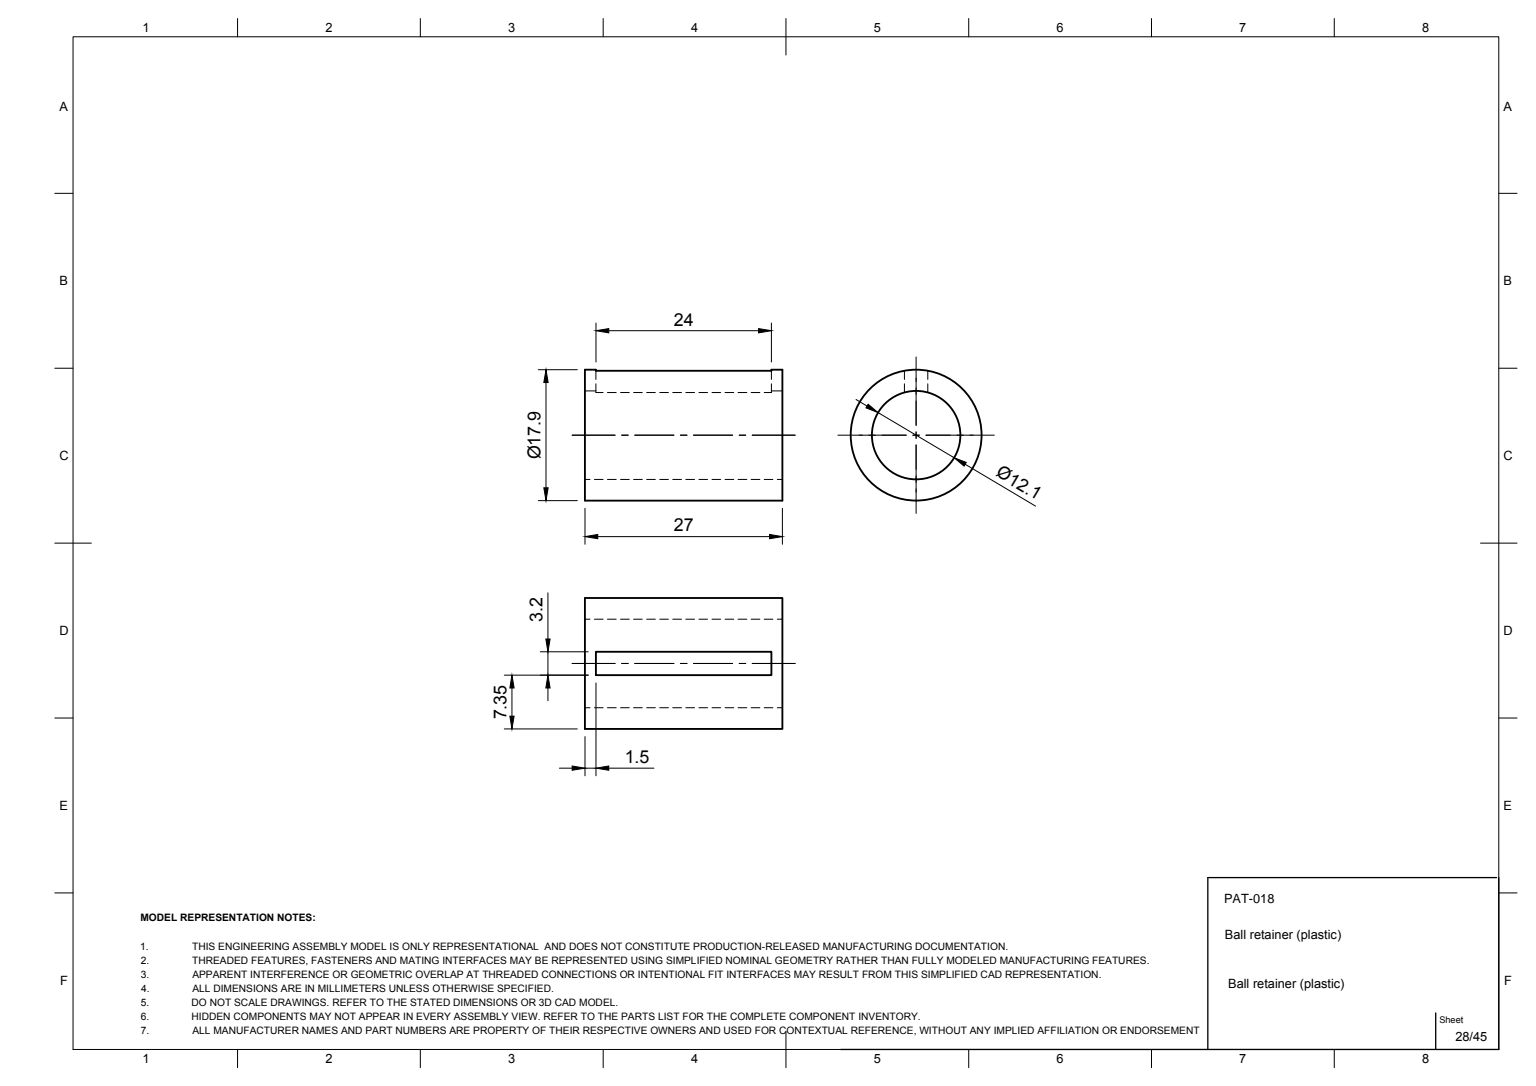
ISO-10303-21;
HEADER;
/* Generated by software containing ST-Developer
 * from STEP Tools, Inc. (www.steptools.com) 
 */

FILE_DESCRIPTION(
/* description */ ('Cam-driven reciprocating slide'),
/* implementation_level */ '2;1');

FILE_NAME(
/* name */ 'Ball retainer (plastic).step',
/* time_stamp */ '2026-10-28T03:25:20-07:00',
/* author */ (''),
/* organization */ (''),
/* preprocessor_version */ 'ST-DEVELOPER v20.2',
/* originating_system */ 'Autodesk Translation Framework v15.17.0.0',
/* authorisation */ '');

FILE_SCHEMA (('AUTOMOTIVE_DESIGN { 1 0 10303 214 3 1 1 }'));
ENDSEC;

DATA;
#10=MECHANICAL_DESIGN_GEOMETRIC_PRESENTATION_REPRESENTATION('',(#449),#13277);
#368=SHAPE_REPRESENTATION_RELATIONSHIP('SRR','None',#13463,#405);
#405=ADVANCED_BREP_SHAPE_REPRESENTATION('',(#492),#13258);
#449=STYLED_ITEM('',(#13713),#492);
#492=MANIFOLD_SOLID_BREP('Body1',#6426);
#635=FACE_BOUND('',#1646,.T.);
#636=FACE_BOUND('',#1648,.T.);
#637=FACE_BOUND('',#1650,.T.);
#638=FACE_BOUND('',#1652,.T.);
#802=PLANE('',#7342);
#803=PLANE('',#7345);
#804=PLANE('',#7346);
#805=PLANE('',#7349);
#806=PLANE('',#7350);
#807=PLANE('',#7355);
#1134=FACE_OUTER_BOUND('',#1641,.T.);
#1135=FACE_OUTER_BOUND('',#1642,.T.);
#1136=FACE_OUTER_BOUND('',#1643,.T.);
#1137=FACE_OUTER_BOUND('',#1644,.T.);
#1138=FACE_OUTER_BOUND('',#1645,.T.);
#1139=FACE_OUTER_BOUND('',#1647,.T.);
#1140=FACE_OUTER_BOUND('',#1649,.T.);
#1141=FACE_OUTER_BOUND('',#1651,.T.);
#1641=EDGE_LOOP('',(#5330,#5331,#5332,#5333));
#1642=EDGE_LOOP('',(#5334,#5335,#5336,#5337));
#1643=EDGE_LOOP('',(#5338,#5339,#5340,#5341));
#1644=EDGE_LOOP('',(#5342,#5343,#5344,#5345));
#1645=EDGE_LOOP('',(#5346));
#1646=EDGE_LOOP('',(#5347));
#1647=EDGE_LOOP('',(#5348,#5349,#5350,#5351));
#1648=EDGE_LOOP('',(#5352,#5353,#5354,#5355));
#1649=EDGE_LOOP('',(#5356));
#1650=EDGE_LOOP('',(#5357));
#1651=EDGE_LOOP('',(#5358,#5359,#5360,#5361));
#1652=EDGE_LOOP('',(#5362,#5363,#5364,#5365));
#2088=LINE('',#12499,#2527);
#2089=LINE('',#12502,#2528);
#2090=LINE('',#12505,#2529);
#2091=LINE('',#12507,#2530);
#2092=LINE('',#12508,#2531);
#2093=LINE('',#12514,#2532);
#2094=LINE('',#12516,#2533);
#2095=LINE('',#12517,#2534);
#2096=LINE('',#12526,#2535);
#2097=LINE('',#12531,#2536);
#2527=VECTOR('',#8906,1.);
#2528=VECTOR('',#8909,1.);
#2529=VECTOR('',#8912,1.);
#2530=VECTOR('',#8913,1.);
#2531=VECTOR('',#8914,1.);
#2532=VECTOR('',#8921,1.);
#2533=VECTOR('',#8924,1.);
#2534=VECTOR('',#8925,1.);
#2535=VECTOR('',#8936,0.895);
#2536=VECTOR('',#8943,0.605);
#2938=CIRCLE('',#7343,0.895);
#2939=CIRCLE('',#7344,0.605);
#2940=CIRCLE('',#7347,0.895);
#2941=CIRCLE('',#7348,0.605);
#2942=CIRCLE('',#7351,0.895);
#2943=CIRCLE('',#7352,0.605);
#2944=CIRCLE('',#7354,0.895);
#2945=CIRCLE('',#7356,0.605);
#3373=VERTEX_POINT('',#12495);
#3374=VERTEX_POINT('',#12496);
#3375=VERTEX_POINT('',#12498);
#3376=VERTEX_POINT('',#12500);
#3377=VERTEX_POINT('',#12504);
#3378=VERTEX_POINT('',#12506);
#3379=VERTEX_POINT('',#12510);
#3380=VERTEX_POINT('',#12512);
#3381=VERTEX_POINT('',#12519);
#3382=VERTEX_POINT('',#12521);
#3383=VERTEX_POINT('',#12524);
#3384=VERTEX_POINT('',#12528);
#4055=EDGE_CURVE('',#3373,#3374,#2938,.T.);
#4056=EDGE_CURVE('',#3375,#3373,#2088,.T.);
#4057=EDGE_CURVE('',#3376,#3375,#2939,.T.);
#4058=EDGE_CURVE('',#3374,#3376,#2089,.T.);
#4059=EDGE_CURVE('',#3374,#3377,#2090,.T.);
#4060=EDGE_CURVE('',#3378,#3376,#2091,.T.);
#4061=EDGE_CURVE('',#3378,#3377,#2092,.T.);
#4062=EDGE_CURVE('',#3377,#3379,#2940,.T.);
#4063=EDGE_CURVE('',#3380,#3378,#2941,.T.);
#4064=EDGE_CURVE('',#3379,#3380,#2093,.T.);
#4065=EDGE_CURVE('',#3379,#3373,#2094,.T.);
#4066=EDGE_CURVE('',#3375,#3380,#2095,.T.);
#4067=EDGE_CURVE('',#3381,#3381,#2942,.T.);
#4068=EDGE_CURVE('',#3382,#3382,#2943,.T.);
#4069=EDGE_CURVE('',#3383,#3383,#2944,.T.);
#4070=EDGE_CURVE('',#3383,#3381,#2096,.T.);
#4071=EDGE_CURVE('',#3384,#3384,#2945,.T.);
#4072=EDGE_CURVE('',#3384,#3382,#2097,.T.);
#5330=ORIENTED_EDGE('',*,*,#4055,.F.);
#5331=ORIENTED_EDGE('',*,*,#4056,.F.);
#5332=ORIENTED_EDGE('',*,*,#4057,.F.);
#5333=ORIENTED_EDGE('',*,*,#4058,.F.);
#5334=ORIENTED_EDGE('',*,*,#4059,.F.);
#5335=ORIENTED_EDGE('',*,*,#4058,.T.);
#5336=ORIENTED_EDGE('',*,*,#4060,.F.);
#5337=ORIENTED_EDGE('',*,*,#4061,.T.);
#5338=ORIENTED_EDGE('',*,*,#4062,.F.);
#5339=ORIENTED_EDGE('',*,*,#4061,.F.);
#5340=ORIENTED_EDGE('',*,*,#4063,.F.);
#5341=ORIENTED_EDGE('',*,*,#4064,.F.);
#5342=ORIENTED_EDGE('',*,*,#4065,.F.);
#5343=ORIENTED_EDGE('',*,*,#4064,.T.);
#5344=ORIENTED_EDGE('',*,*,#4066,.F.);
#5345=ORIENTED_EDGE('',*,*,#4056,.T.);
#5346=ORIENTED_EDGE('',*,*,#4067,.F.);
#5347=ORIENTED_EDGE('',*,*,#4068,.T.);
#5348=ORIENTED_EDGE('',*,*,#4069,.F.);
#5349=ORIENTED_EDGE('',*,*,#4070,.T.);
#5350=ORIENTED_EDGE('',*,*,#4067,.T.);
#5351=ORIENTED_EDGE('',*,*,#4070,.F.);
#5352=ORIENTED_EDGE('',*,*,#4062,.T.);
#5353=ORIENTED_EDGE('',*,*,#4065,.T.);
#5354=ORIENTED_EDGE('',*,*,#4055,.T.);
#5355=ORIENTED_EDGE('',*,*,#4059,.T.);
#5356=ORIENTED_EDGE('',*,*,#4069,.T.);
#5357=ORIENTED_EDGE('',*,*,#4071,.F.);
#5358=ORIENTED_EDGE('',*,*,#4071,.T.);
#5359=ORIENTED_EDGE('',*,*,#4072,.T.);
#5360=ORIENTED_EDGE('',*,*,#4068,.F.);
#5361=ORIENTED_EDGE('',*,*,#4072,.F.);
#5362=ORIENTED_EDGE('',*,*,#4063,.T.);
#5363=ORIENTED_EDGE('',*,*,#4060,.T.);
#5364=ORIENTED_EDGE('',*,*,#4057,.T.);
#5365=ORIENTED_EDGE('',*,*,#4066,.T.);
#5979=CYLINDRICAL_SURFACE('',#7353,0.895);
#5980=CYLINDRICAL_SURFACE('',#7357,0.605);
#6252=ADVANCED_FACE('',(#1134),#802,.F.);
#6253=ADVANCED_FACE('',(#1135),#803,.F.);
#6254=ADVANCED_FACE('',(#1136),#804,.F.);
#6255=ADVANCED_FACE('',(#1137),#805,.F.);
#6256=ADVANCED_FACE('',(#1138,#635),#806,.T.);
#6257=ADVANCED_FACE('',(#1139,#636),#5979,.T.);
#6258=ADVANCED_FACE('',(#1140,#637),#807,.T.);
#6259=ADVANCED_FACE('',(#1141,#638),#5980,.F.);
#6426=CLOSED_SHELL('',(#6252,#6253,#6254,#6255,#6256,#6257,#6258,#6259));
#7341=AXIS2_PLACEMENT_3D('',#12493,#8900,#8901);
#7342=AXIS2_PLACEMENT_3D('',#12494,#8902,#8903);
#7343=AXIS2_PLACEMENT_3D('',#12497,#8904,#8905);
#7344=AXIS2_PLACEMENT_3D('',#12501,#8907,#8908);
#7345=AXIS2_PLACEMENT_3D('',#12503,#8910,#8911);
#7346=AXIS2_PLACEMENT_3D('',#12509,#8915,#8916);
#7347=AXIS2_PLACEMENT_3D('',#12511,#8917,#8918);
#7348=AXIS2_PLACEMENT_3D('',#12513,#8919,#8920);
#7349=AXIS2_PLACEMENT_3D('',#12515,#8922,#8923);
#7350=AXIS2_PLACEMENT_3D('',#12518,#8926,#8927);
#7351=AXIS2_PLACEMENT_3D('',#12520,#8928,#8929);
#7352=AXIS2_PLACEMENT_3D('',#12522,#8930,#8931);
#7353=AXIS2_PLACEMENT_3D('',#12523,#8932,#8933);
#7354=AXIS2_PLACEMENT_3D('',#12525,#8934,#8935);
#7355=AXIS2_PLACEMENT_3D('',#12527,#8937,#8938);
#7356=AXIS2_PLACEMENT_3D('',#12529,#8939,#8940);
#7357=AXIS2_PLACEMENT_3D('',#12530,#8941,#8942);
#8900=DIRECTION('axis',(0.,0.,1.));
#8901=DIRECTION('refdir',(1.,0.,0.));
#8902=DIRECTION('center_axis',(0.,1.,0.));
#8903=DIRECTION('ref_axis',(0.,0.,1.));
#8904=DIRECTION('center_axis',(0.,1.,0.));
#8905=DIRECTION('ref_axis',(1.,0.,0.));
#8906=DIRECTION('',(1.,0.,0.));
#8907=DIRECTION('center_axis',(0.,-1.,0.));
#8908=DIRECTION('ref_axis',(1.,0.,0.));
#8909=DIRECTION('',(-1.,0.,0.));
#8910=DIRECTION('center_axis',(0.,0.,-1.));
#8911=DIRECTION('ref_axis',(-1.,0.,0.));
#8912=DIRECTION('',(0.,-1.,0.));
#8913=DIRECTION('',(0.,1.,0.));
#8914=DIRECTION('',(1.,0.,0.));
#8915=DIRECTION('center_axis',(0.,-1.,0.));
#8916=DIRECTION('ref_axis',(0.,0.,-1.));
#8917=DIRECTION('center_axis',(0.,-1.,0.));
#8918=DIRECTION('ref_axis',(1.,0.,0.));
#8919=DIRECTION('center_axis',(0.,1.,0.));
#8920=DIRECTION('ref_axis',(1.,0.,0.));
#8921=DIRECTION('',(-1.,0.,0.));
#8922=DIRECTION('center_axis',(0.,0.,1.));
#8923=DIRECTION('ref_axis',(1.,0.,0.));
#8924=DIRECTION('',(0.,1.,0.));
#8925=DIRECTION('',(0.,-1.,0.));
#8926=DIRECTION('center_axis',(0.,1.,0.));
#8927=DIRECTION('ref_axis',(0.,0.,1.));
#8928=DIRECTION('center_axis',(0.,-1.,0.));
#8929=DIRECTION('ref_axis',(1.,0.,0.));
#8930=DIRECTION('center_axis',(0.,-1.,0.));
#8931=DIRECTION('ref_axis',(1.,0.,0.));
#8932=DIRECTION('center_axis',(0.,-1.,0.));
#8933=DIRECTION('ref_axis',(1.,0.,0.));
#8934=DIRECTION('center_axis',(0.,-1.,0.));
#8935=DIRECTION('ref_axis',(1.,0.,0.));
#8936=DIRECTION('',(0.,1.,0.));
#8937=DIRECTION('center_axis',(0.,-1.,0.));
#8938=DIRECTION('ref_axis',(0.,0.,-1.));
#8939=DIRECTION('center_axis',(0.,-1.,0.));
#8940=DIRECTION('ref_axis',(1.,0.,0.));
#8941=DIRECTION('center_axis',(0.,-1.,0.));
#8942=DIRECTION('ref_axis',(1.,0.,0.));
#8943=DIRECTION('',(0.,1.,0.));
#12493=CARTESIAN_POINT('',(0.,0.,0.));
#12494=CARTESIAN_POINT('Origin',(0.75,1.2,0.));
#12495=CARTESIAN_POINT('',(0.880582193778639,1.2,0.16));
#12496=CARTESIAN_POINT('',(0.880582193778639,1.2,-0.16));
#12497=CARTESIAN_POINT('Origin',(0.,1.2,0.));
#12498=CARTESIAN_POINT('',(0.583459510163302,1.2,0.16));
#12499=CARTESIAN_POINT('',(0.57,1.2,0.16));
#12500=CARTESIAN_POINT('',(0.583459510163302,1.2,-0.16));
#12501=CARTESIAN_POINT('Origin',(0.,1.2,0.));
#12502=CARTESIAN_POINT('',(0.93,1.2,-0.16));
#12503=CARTESIAN_POINT('Origin',(0.93,0.,-0.16));
#12504=CARTESIAN_POINT('',(0.880582193778639,-1.2,-0.16));
#12505=CARTESIAN_POINT('',(0.880582193778639,0.,-0.16));
#12506=CARTESIAN_POINT('',(0.583459510163302,-1.2,-0.16));
#12507=CARTESIAN_POINT('',(0.583459510163302,0.,-0.16));
#12508=CARTESIAN_POINT('',(0.93,-1.2,-0.16));
#12509=CARTESIAN_POINT('Origin',(0.75,-1.2,0.));
#12510=CARTESIAN_POINT('',(0.880582193778639,-1.2,0.16));
#12511=CARTESIAN_POINT('Origin',(0.,-1.2,0.));
#12512=CARTESIAN_POINT('',(0.583459510163302,-1.2,0.16));
#12513=CARTESIAN_POINT('Origin',(0.,-1.2,0.));
#12514=CARTESIAN_POINT('',(0.57,-1.2,0.16));
#12515=CARTESIAN_POINT('Origin',(0.57,0.,0.16));
#12516=CARTESIAN_POINT('',(0.880582193778639,0.,0.16));
#12517=CARTESIAN_POINT('',(0.583459510163302,0.,0.16));
#12518=CARTESIAN_POINT('Origin',(0.895,1.35,0.));
#12519=CARTESIAN_POINT('',(-0.895,1.35,-1.09605888523688E-16));
#12520=CARTESIAN_POINT('Origin',(0.,1.35,0.));
#12521=CARTESIAN_POINT('',(-0.605,1.35,-7.40911313484149E-17));
#12522=CARTESIAN_POINT('Origin',(0.,1.35,0.));
#12523=CARTESIAN_POINT('Origin',(0.,0.,0.));
#12524=CARTESIAN_POINT('',(-0.895,-1.35,-1.09605888523688E-16));
#12525=CARTESIAN_POINT('Origin',(0.,-1.35,0.));
#12526=CARTESIAN_POINT('',(-0.895,0.,-1.09605888523688E-16));
#12527=CARTESIAN_POINT('Origin',(0.605,-1.35,0.));
#12528=CARTESIAN_POINT('',(-0.605,-1.35,-7.40911313484149E-17));
#12529=CARTESIAN_POINT('Origin',(0.,-1.35,0.));
#12530=CARTESIAN_POINT('Origin',(0.,0.,0.));
#12531=CARTESIAN_POINT('',(-0.605,0.,-7.40911313484149E-17));
#13214=UNCERTAINTY_MEASURE_WITH_UNIT(LENGTH_MEASURE(0.001),#13278,
'DISTANCE_ACCURACY_VALUE',
'Maximum model space distance between geometric entities at asserted c
onnectivities');
#13233=UNCERTAINTY_MEASURE_WITH_UNIT(LENGTH_MEASURE(0.001),#13278,
'DISTANCE_ACCURACY_VALUE',
'Maximum model space distance between geometric entities at asserted c
onnectivities');
#13258=(
GEOMETRIC_REPRESENTATION_CONTEXT(3)
GLOBAL_UNCERTAINTY_ASSIGNED_CONTEXT((#13214))
GLOBAL_UNIT_ASSIGNED_CONTEXT((#13278,#13280,#13281))
REPRESENTATION_CONTEXT('','3D')
);
#13277=(
GEOMETRIC_REPRESENTATION_CONTEXT(3)
GLOBAL_UNCERTAINTY_ASSIGNED_CONTEXT((#13233))
GLOBAL_UNIT_ASSIGNED_CONTEXT((#13278,#13280,#13281))
REPRESENTATION_CONTEXT('','3D')
);
#13278=(
LENGTH_UNIT()
NAMED_UNIT(*)
SI_UNIT(.CENTI.,.METRE.)
);
#13280=(
NAMED_UNIT(*)
PLANE_ANGLE_UNIT()
SI_UNIT($,.RADIAN.)
);
#13281=(
NAMED_UNIT(*)
SI_UNIT($,.STERADIAN.)
SOLID_ANGLE_UNIT()
);
#13306=SHAPE_DEFINITION_REPRESENTATION(#13354,#13463);
#13354=PRODUCT_DEFINITION_SHAPE('',$,#13507);
#13463=SHAPE_REPRESENTATION('',(#7341),#13258);
#13482=PRODUCT_DEFINITION_CONTEXT('part definition',#13613,'design');
#13507=PRODUCT_DEFINITION('Ball retainer (plastic)',
'Ball retainer (plastic)',#13550,#13482);
#13550=PRODUCT_DEFINITION_FORMATION('',$,#13639);
#13613=APPLICATION_CONTEXT(
'Core Data for Automotive Mechanical Design Process');
#13614=PRODUCT_CONTEXT('part definition',#13613,'mechanical');
#13639=PRODUCT('Ball retainer (plastic)','Ball retainer (plastic)',
'Ball retainer (plastic)',(#13614));
#13707=COLOUR_RGB('Sky Blue',0.24,0.69,0.87);
#13708=FILL_AREA_STYLE_COLOUR('',#13707);
#13709=FILL_AREA_STYLE('',(#13708));
#13710=SURFACE_STYLE_FILL_AREA(#13709);
#13711=SURFACE_SIDE_STYLE('',(#13710));
#13712=SURFACE_STYLE_USAGE(.BOTH.,#13711);
#13713=PRESENTATION_STYLE_ASSIGNMENT((#13712));
ENDSEC;
END-ISO-10303-21;
